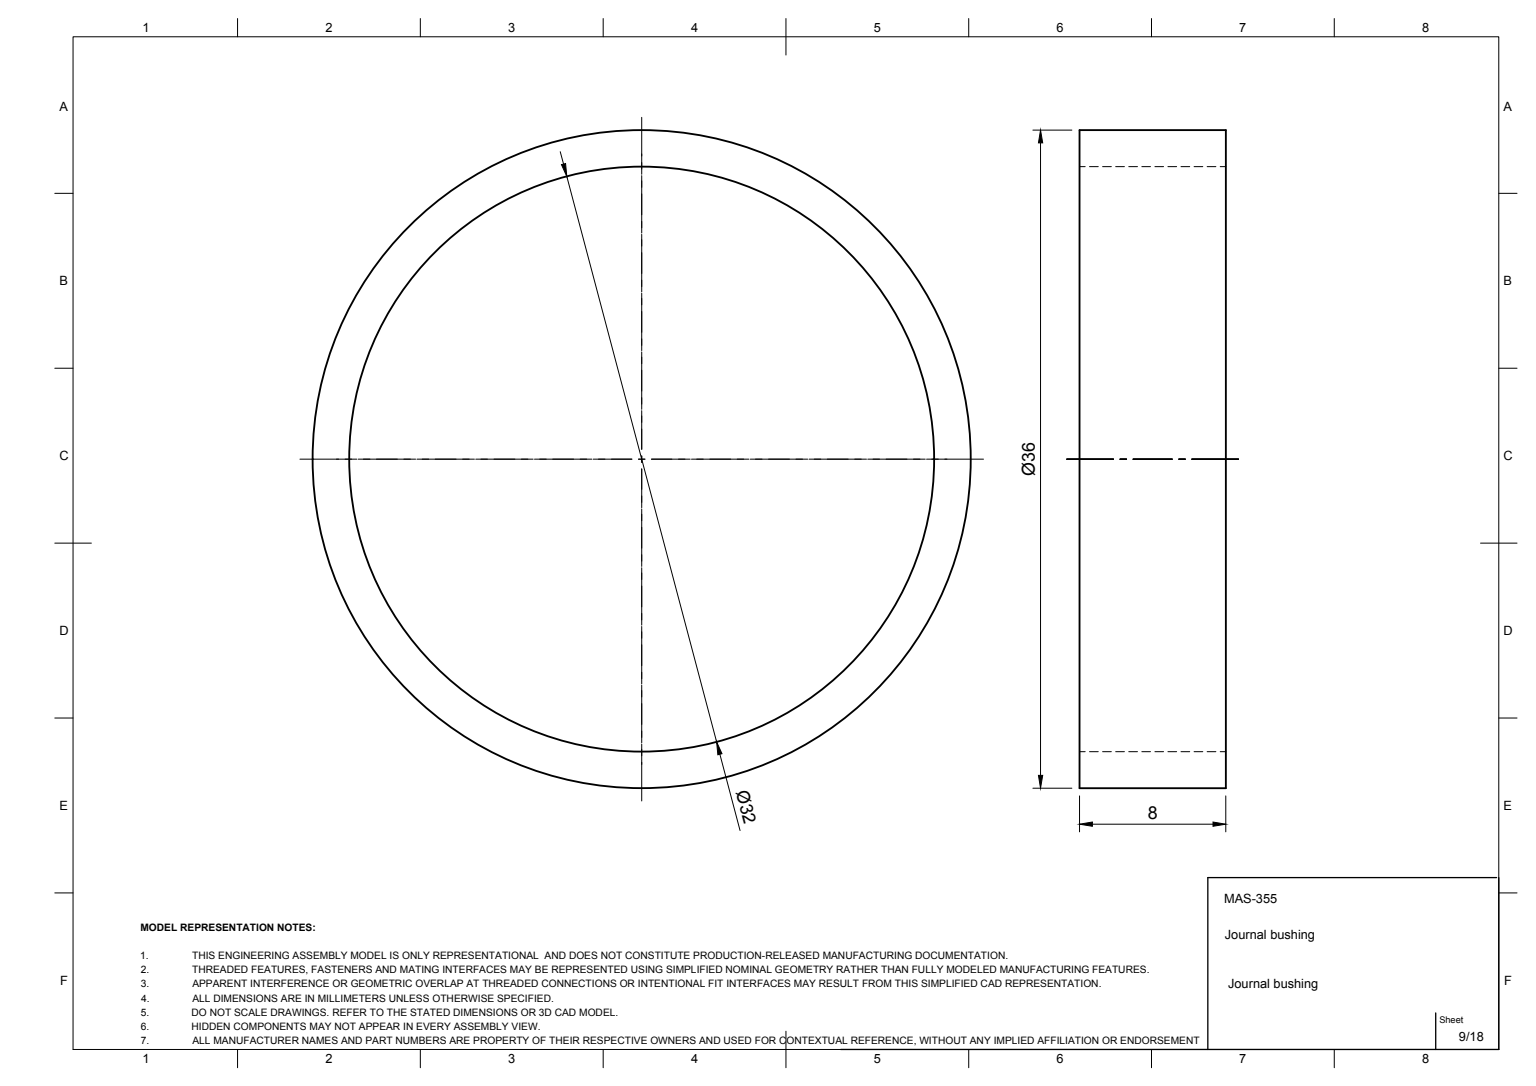
ISO-10303-21;
HEADER;
/* Generated by software containing ST-Developer
 * from STEP Tools, Inc. (www.steptools.com) 
 */

FILE_DESCRIPTION(
/* description */ ('Independent two-stage fixed-ring planetary gearbox,24/24/72 teeth,mod
ule2,20deg involutes,three planets per stage,4:1 x4:1=16:1. Native cut
-space/fillet/pattern tooth profiles derived from reusable gear blanks
; shared sun/planet/ring/carrier parts across both stages. Captured br
onze-journal input/carriers, headed retained planet pins, keyed inters
tage drive and modular keyed output interface. Native ideal gear links
; no torque, precision grade, production backlash/fits, lubrication, s
peed or life rating.'),
/* implementation_level */ '2;1');

FILE_NAME(
/* name */ 'Journal bushing.step',
/* time_stamp */ '2026-11-08T19:10:00-08:00',
/* author */ (''),
/* organization */ (''),
/* preprocessor_version */ 'ST-DEVELOPER v20.2',
/* originating_system */ 'Autodesk Translation Framework v15.17.0.0',
/* authorisation */ '');

FILE_SCHEMA (('AUTOMOTIVE_DESIGN { 1 0 10303 214 3 1 1 }'));
ENDSEC;

DATA;
#10=MECHANICAL_DESIGN_GEOMETRIC_PRESENTATION_REPRESENTATION('',(#1170),#259224);
#1130=SHAPE_REPRESENTATION_RELATIONSHIP('SRR','None',#259377,#1150);
#1150=ADVANCED_BREP_SHAPE_REPRESENTATION('',(#1190),#259211);
#1170=STYLED_ITEM('',(#259485),#1190);
#1190=MANIFOLD_SOLID_BREP('Body1',#25157);
#1285=FACE_BOUND('',#4331,.T.);
#1286=FACE_BOUND('',#4333,.T.);
#1635=PLANE('',#27008);
#1636=PLANE('',#27009);
#2900=FACE_OUTER_BOUND('',#4328,.T.);
#2901=FACE_OUTER_BOUND('',#4329,.T.);
#2902=FACE_OUTER_BOUND('',#4330,.T.);
#2903=FACE_OUTER_BOUND('',#4332,.T.);
#4328=EDGE_LOOP('',(#22472,#22473,#22474,#22475));
#4329=EDGE_LOOP('',(#22476,#22477,#22478,#22479));
#4330=EDGE_LOOP('',(#22480));
#4331=EDGE_LOOP('',(#22481));
#4332=EDGE_LOOP('',(#22482));
#4333=EDGE_LOOP('',(#22483));
#5305=CIRCLE('',#27003,16.);
#5306=CIRCLE('',#27004,16.);
#5307=CIRCLE('',#27006,18.);
#5308=CIRCLE('',#27007,18.);
#7717=LINE('',#255762,#8902);
#7718=LINE('',#255768,#8903);
#8902=VECTOR('',#31610,16.);
#8903=VECTOR('',#31617,18.);
#11395=VERTEX_POINT('',#255759);
#11396=VERTEX_POINT('',#255761);
#11397=VERTEX_POINT('',#255765);
#11398=VERTEX_POINT('',#255767);
#15121=EDGE_CURVE('',#11395,#11395,#5305,.T.);
#15122=EDGE_CURVE('',#11395,#11396,#7717,.T.);
#15123=EDGE_CURVE('',#11396,#11396,#5306,.T.);
#15124=EDGE_CURVE('',#11397,#11397,#5307,.T.);
#15125=EDGE_CURVE('',#11397,#11398,#7718,.T.);
#15126=EDGE_CURVE('',#11398,#11398,#5308,.T.);
#22472=ORIENTED_EDGE('',*,*,#15121,.F.);
#22473=ORIENTED_EDGE('',*,*,#15122,.T.);
#22474=ORIENTED_EDGE('',*,*,#15123,.T.);
#22475=ORIENTED_EDGE('',*,*,#15122,.F.);
#22476=ORIENTED_EDGE('',*,*,#15124,.F.);
#22477=ORIENTED_EDGE('',*,*,#15125,.T.);
#22478=ORIENTED_EDGE('',*,*,#15126,.T.);
#22479=ORIENTED_EDGE('',*,*,#15125,.F.);
#22480=ORIENTED_EDGE('',*,*,#15124,.T.);
#22481=ORIENTED_EDGE('',*,*,#15121,.T.);
#22482=ORIENTED_EDGE('',*,*,#15126,.F.);
#22483=ORIENTED_EDGE('',*,*,#15123,.F.);
#23725=CYLINDRICAL_SURFACE('',#27002,16.);
#23726=CYLINDRICAL_SURFACE('',#27005,18.);
#25006=ADVANCED_FACE('',(#2900),#23725,.F.);
#25007=ADVANCED_FACE('',(#2901),#23726,.T.);
#25008=ADVANCED_FACE('',(#2902,#1285),#1635,.T.);
#25009=ADVANCED_FACE('',(#2903,#1286),#1636,.F.);
#25157=CLOSED_SHELL('',(#25006,#25007,#25008,#25009));
#27001=AXIS2_PLACEMENT_3D('',#255757,#31604,#31605);
#27002=AXIS2_PLACEMENT_3D('',#255758,#31606,#31607);
#27003=AXIS2_PLACEMENT_3D('',#255760,#31608,#31609);
#27004=AXIS2_PLACEMENT_3D('',#255763,#31611,#31612);
#27005=AXIS2_PLACEMENT_3D('',#255764,#31613,#31614);
#27006=AXIS2_PLACEMENT_3D('',#255766,#31615,#31616);
#27007=AXIS2_PLACEMENT_3D('',#255769,#31618,#31619);
#27008=AXIS2_PLACEMENT_3D('',#255770,#31620,#31621);
#27009=AXIS2_PLACEMENT_3D('',#255771,#31622,#31623);
#31604=DIRECTION('axis',(0.,0.,1.));
#31605=DIRECTION('refdir',(1.,0.,0.));
#31606=DIRECTION('center_axis',(0.,0.,1.));
#31607=DIRECTION('ref_axis',(1.,0.,0.));
#31608=DIRECTION('center_axis',(0.,0.,-1.));
#31609=DIRECTION('ref_axis',(1.,0.,0.));
#31610=DIRECTION('',(0.,0.,-1.));
#31611=DIRECTION('center_axis',(0.,0.,-1.));
#31612=DIRECTION('ref_axis',(1.,0.,0.));
#31613=DIRECTION('center_axis',(0.,0.,1.));
#31614=DIRECTION('ref_axis',(1.,0.,0.));
#31615=DIRECTION('center_axis',(0.,0.,1.));
#31616=DIRECTION('ref_axis',(1.,0.,0.));
#31617=DIRECTION('',(0.,0.,-1.));
#31618=DIRECTION('center_axis',(0.,0.,1.));
#31619=DIRECTION('ref_axis',(1.,0.,0.));
#31620=DIRECTION('center_axis',(0.,0.,1.));
#31621=DIRECTION('ref_axis',(1.,0.,0.));
#31622=DIRECTION('center_axis',(0.,0.,1.));
#31623=DIRECTION('ref_axis',(1.,0.,0.));
#255757=CARTESIAN_POINT('',(0.,0.,0.));
#255758=CARTESIAN_POINT('Origin',(0.,0.,0.));
#255759=CARTESIAN_POINT('',(-16.,-1.95943487863577E-15,8.));
#255760=CARTESIAN_POINT('Origin',(0.,0.,8.));
#255761=CARTESIAN_POINT('',(-16.,-1.95943487863577E-15,0.));
#255762=CARTESIAN_POINT('',(-16.,-1.95943487863577E-15,0.));
#255763=CARTESIAN_POINT('Origin',(0.,0.,0.));
#255764=CARTESIAN_POINT('Origin',(0.,0.,0.));
#255765=CARTESIAN_POINT('',(-18.,-2.20436423846524E-15,8.));
#255766=CARTESIAN_POINT('Origin',(0.,0.,8.));
#255767=CARTESIAN_POINT('',(-18.,-2.20436423846524E-15,0.));
#255768=CARTESIAN_POINT('',(-18.,-2.20436423846524E-15,0.));
#255769=CARTESIAN_POINT('Origin',(0.,0.,0.));
#255770=CARTESIAN_POINT('Origin',(0.,0.,8.));
#255771=CARTESIAN_POINT('Origin',(0.,0.,0.));
#259189=UNCERTAINTY_MEASURE_WITH_UNIT(LENGTH_MEASURE(0.01),#259225,
'DISTANCE_ACCURACY_VALUE',
'Maximum model space distance between geometric entities at asserted c
onnectivities');
#259202=UNCERTAINTY_MEASURE_WITH_UNIT(LENGTH_MEASURE(0.01),#259225,
'DISTANCE_ACCURACY_VALUE',
'Maximum model space distance between geometric entities at asserted c
onnectivities');
#259211=(
GEOMETRIC_REPRESENTATION_CONTEXT(3)
GLOBAL_UNCERTAINTY_ASSIGNED_CONTEXT((#259189))
GLOBAL_UNIT_ASSIGNED_CONTEXT((#259225,#259227,#259228))
REPRESENTATION_CONTEXT('','3D')
);
#259224=(
GEOMETRIC_REPRESENTATION_CONTEXT(3)
GLOBAL_UNCERTAINTY_ASSIGNED_CONTEXT((#259202))
GLOBAL_UNIT_ASSIGNED_CONTEXT((#259225,#259227,#259228))
REPRESENTATION_CONTEXT('','3D')
);
#259225=(
LENGTH_UNIT()
NAMED_UNIT(*)
SI_UNIT(.MILLI.,.METRE.)
);
#259227=(
NAMED_UNIT(*)
PLANE_ANGLE_UNIT()
SI_UNIT($,.RADIAN.)
);
#259228=(
NAMED_UNIT(*)
SI_UNIT($,.STERADIAN.)
SOLID_ANGLE_UNIT()
);
#259237=SHAPE_DEFINITION_REPRESENTATION(#259258,#259377);
#259258=PRODUCT_DEFINITION_SHAPE('',$,#259399);
#259377=SHAPE_REPRESENTATION('',(#27001),#259211);
#259390=PRODUCT_DEFINITION_CONTEXT('part definition',#259455,'design');
#259399=PRODUCT_DEFINITION('Journal bushing','Journal bushing',#259420,
#259390);
#259420=PRODUCT_DEFINITION_FORMATION('',$,#259465);
#259455=APPLICATION_CONTEXT(
'Core Data for Automotive Mechanical Design Process');
#259456=PRODUCT_CONTEXT('part definition',#259455,'mechanical');
#259465=PRODUCT('Journal bushing','Journal bushing',$,(#259456));
#259485=PRESENTATION_STYLE_ASSIGNMENT((#259500));
#259500=SURFACE_STYLE_USAGE(.BOTH.,#259515);
#259515=SURFACE_SIDE_STYLE('',(#259530));
#259530=SURFACE_STYLE_FILL_AREA(#259545);
#259545=FILL_AREA_STYLE('Bearing light gray',(#259560));
#259560=FILL_AREA_STYLE_COLOUR('Bearing light gray',#259575);
#259575=COLOUR_RGB('Bearing light gray',0.725490196078431,0.752941176470588,
0.792156862745098);
ENDSEC;
END-ISO-10303-21;
